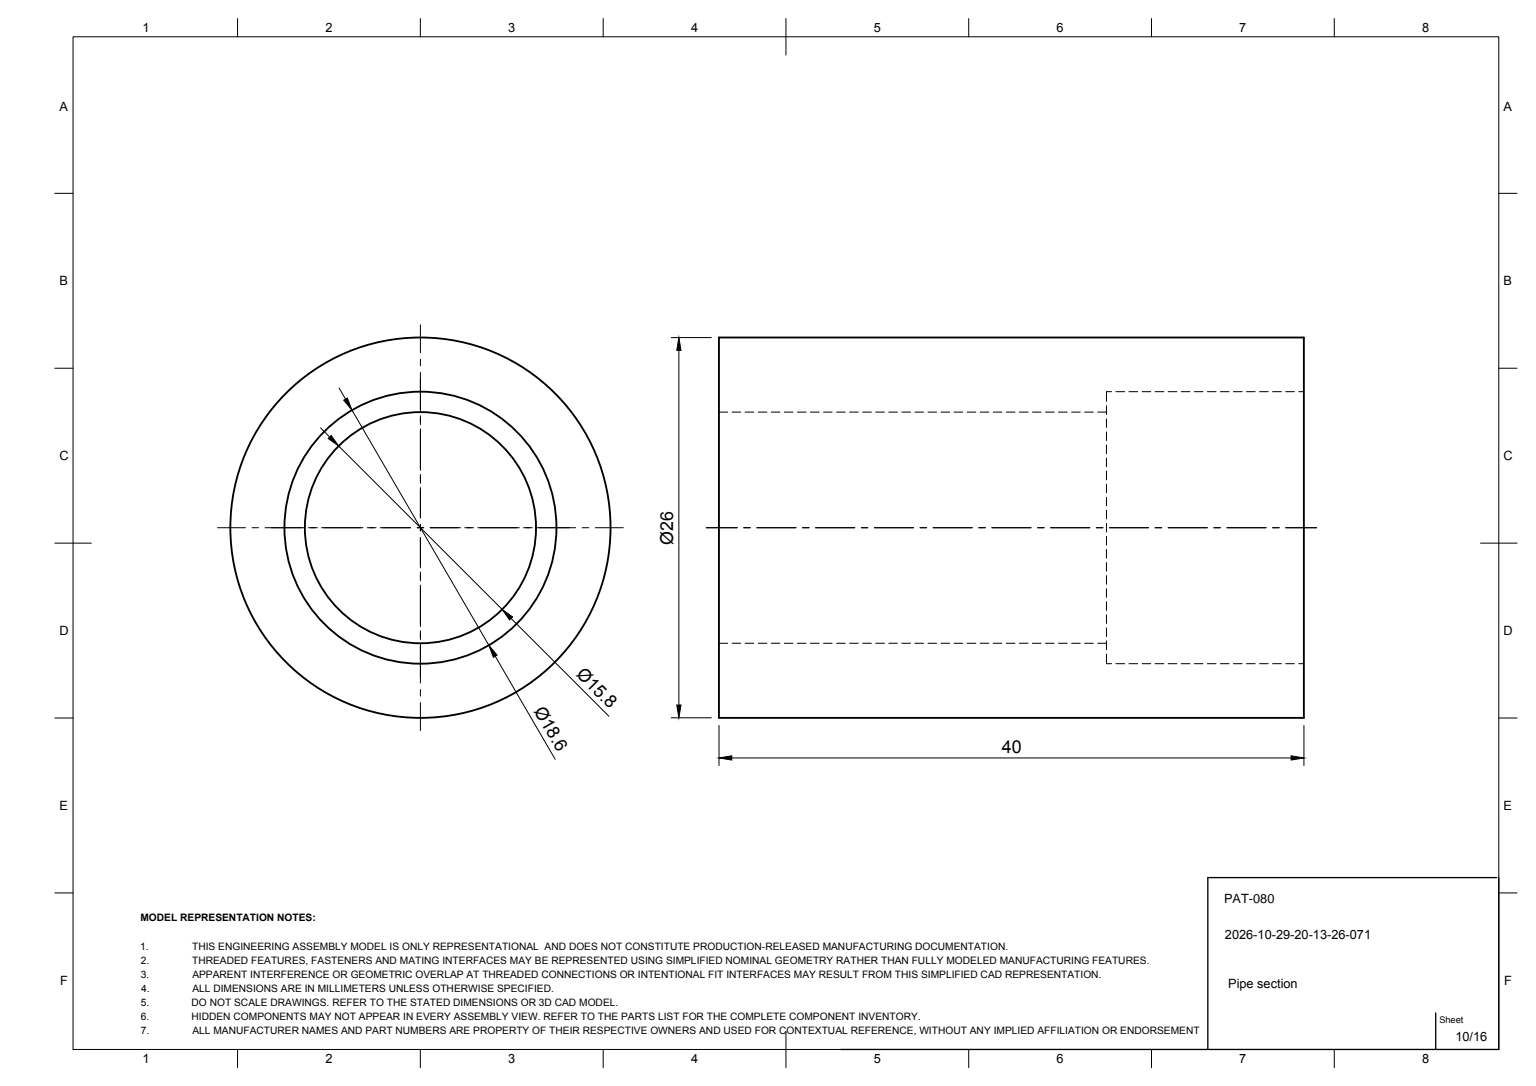
ISO-10303-21;
HEADER;
/* Generated by software containing ST-Developer
 * from STEP Tools, Inc. (www.steptools.com) 
 */

FILE_DESCRIPTION(
/* description */ ('PAT-080'),
/* implementation_level */ '2;1');

FILE_NAME(
/* name */ 'Pipe section.step',
/* time_stamp */ '2026-10-29T20:13:47-07:00',
/* author */ (''),
/* organization */ (''),
/* preprocessor_version */ 'ST-DEVELOPER v20.2',
/* originating_system */ 'Autodesk Translation Framework v15.17.0.0',
/* authorisation */ '');

FILE_SCHEMA (('AUTOMOTIVE_DESIGN { 1 0 10303 214 3 1 1 }'));
ENDSEC;

DATA;
#10=MECHANICAL_DESIGN_GEOMETRIC_PRESENTATION_REPRESENTATION('',(#253),#6878);
#215=SHAPE_REPRESENTATION_RELATIONSHIP('SRR','None',#6971,#234);
#234=ADVANCED_BREP_SHAPE_REPRESENTATION('',(#272),#6866);
#253=STYLED_ITEM('',(#7122),#272);
#272=MANIFOLD_SOLID_BREP('Body1',#3869);
#309=FACE_BOUND('',#850,.T.);
#310=FACE_BOUND('',#854,.T.);
#311=FACE_BOUND('',#856,.T.);
#427=PLANE('',#4248);
#428=PLANE('',#4255);
#429=PLANE('',#4256);
#594=FACE_OUTER_BOUND('',#848,.T.);
#595=FACE_OUTER_BOUND('',#849,.T.);
#596=FACE_OUTER_BOUND('',#851,.T.);
#597=FACE_OUTER_BOUND('',#852,.T.);
#598=FACE_OUTER_BOUND('',#853,.T.);
#599=FACE_OUTER_BOUND('',#855,.T.);
#848=EDGE_LOOP('',(#3064,#3065,#3066,#3067));
#849=EDGE_LOOP('',(#3068));
#850=EDGE_LOOP('',(#3069));
#851=EDGE_LOOP('',(#3070,#3071,#3072,#3073));
#852=EDGE_LOOP('',(#3074,#3075,#3076,#3077));
#853=EDGE_LOOP('',(#3078));
#854=EDGE_LOOP('',(#3079));
#855=EDGE_LOOP('',(#3080));
#856=EDGE_LOOP('',(#3081));
#1208=LINE('',#6216,#1523);
#1209=LINE('',#6224,#1524);
#1210=LINE('',#6229,#1525);
#1523=VECTOR('',#5020,0.93);
#1524=VECTOR('',#5031,0.79);
#1525=VECTOR('',#5036,1.3);
#1706=CIRCLE('',#4246,0.93);
#1707=CIRCLE('',#4247,0.93);
#1708=CIRCLE('',#4249,0.79);
#1709=CIRCLE('',#4251,0.79);
#1710=CIRCLE('',#4253,1.3);
#1711=CIRCLE('',#4254,1.3);
#1962=VERTEX_POINT('',#6213);
#1963=VERTEX_POINT('',#6215);
#1964=VERTEX_POINT('',#6219);
#1965=VERTEX_POINT('',#6222);
#1966=VERTEX_POINT('',#6226);
#1967=VERTEX_POINT('',#6228);
#2355=EDGE_CURVE('',#1962,#1962,#1706,.T.);
#2356=EDGE_CURVE('',#1962,#1963,#1208,.T.);
#2357=EDGE_CURVE('',#1963,#1963,#1707,.T.);
#2358=EDGE_CURVE('',#1964,#1964,#1708,.T.);
#2359=EDGE_CURVE('',#1965,#1965,#1709,.T.);
#2360=EDGE_CURVE('',#1965,#1964,#1209,.T.);
#2361=EDGE_CURVE('',#1966,#1966,#1710,.T.);
#2362=EDGE_CURVE('',#1966,#1967,#1210,.T.);
#2363=EDGE_CURVE('',#1967,#1967,#1711,.T.);
#3064=ORIENTED_EDGE('',*,*,#2355,.F.);
#3065=ORIENTED_EDGE('',*,*,#2356,.T.);
#3066=ORIENTED_EDGE('',*,*,#2357,.T.);
#3067=ORIENTED_EDGE('',*,*,#2356,.F.);
#3068=ORIENTED_EDGE('',*,*,#2357,.F.);
#3069=ORIENTED_EDGE('',*,*,#2358,.F.);
#3070=ORIENTED_EDGE('',*,*,#2359,.F.);
#3071=ORIENTED_EDGE('',*,*,#2360,.T.);
#3072=ORIENTED_EDGE('',*,*,#2358,.T.);
#3073=ORIENTED_EDGE('',*,*,#2360,.F.);
#3074=ORIENTED_EDGE('',*,*,#2361,.F.);
#3075=ORIENTED_EDGE('',*,*,#2362,.T.);
#3076=ORIENTED_EDGE('',*,*,#2363,.T.);
#3077=ORIENTED_EDGE('',*,*,#2362,.F.);
#3078=ORIENTED_EDGE('',*,*,#2361,.T.);
#3079=ORIENTED_EDGE('',*,*,#2359,.T.);
#3080=ORIENTED_EDGE('',*,*,#2363,.F.);
#3081=ORIENTED_EDGE('',*,*,#2355,.T.);
#3594=CYLINDRICAL_SURFACE('',#4245,0.93);
#3595=CYLINDRICAL_SURFACE('',#4250,0.79);
#3596=CYLINDRICAL_SURFACE('',#4252,1.3);
#3730=ADVANCED_FACE('',(#594),#3594,.F.);
#3731=ADVANCED_FACE('',(#595,#309),#427,.F.);
#3732=ADVANCED_FACE('',(#596),#3595,.F.);
#3733=ADVANCED_FACE('',(#597),#3596,.T.);
#3734=ADVANCED_FACE('',(#598,#310),#428,.T.);
#3735=ADVANCED_FACE('',(#599,#311),#429,.F.);
#3869=CLOSED_SHELL('',(#3730,#3731,#3732,#3733,#3734,#3735));
#4244=AXIS2_PLACEMENT_3D('',#6211,#5014,#5015);
#4245=AXIS2_PLACEMENT_3D('',#6212,#5016,#5017);
#4246=AXIS2_PLACEMENT_3D('',#6214,#5018,#5019);
#4247=AXIS2_PLACEMENT_3D('',#6217,#5021,#5022);
#4248=AXIS2_PLACEMENT_3D('',#6218,#5023,#5024);
#4249=AXIS2_PLACEMENT_3D('',#6220,#5025,#5026);
#4250=AXIS2_PLACEMENT_3D('',#6221,#5027,#5028);
#4251=AXIS2_PLACEMENT_3D('',#6223,#5029,#5030);
#4252=AXIS2_PLACEMENT_3D('',#6225,#5032,#5033);
#4253=AXIS2_PLACEMENT_3D('',#6227,#5034,#5035);
#4254=AXIS2_PLACEMENT_3D('',#6230,#5037,#5038);
#4255=AXIS2_PLACEMENT_3D('',#6231,#5039,#5040);
#4256=AXIS2_PLACEMENT_3D('',#6232,#5041,#5042);
#5014=DIRECTION('axis',(0.,0.,1.));
#5015=DIRECTION('refdir',(1.,0.,0.));
#5016=DIRECTION('center_axis',(1.,0.,0.));
#5017=DIRECTION('ref_axis',(0.,0.,-1.));
#5018=DIRECTION('center_axis',(1.,0.,0.));
#5019=DIRECTION('ref_axis',(0.,0.,-1.));
#5020=DIRECTION('',(1.,0.,0.));
#5021=DIRECTION('center_axis',(1.,0.,0.));
#5022=DIRECTION('ref_axis',(0.,0.,-1.));
#5023=DIRECTION('center_axis',(1.,0.,0.));
#5024=DIRECTION('ref_axis',(0.,0.,-1.));
#5025=DIRECTION('center_axis',(-1.,0.,0.));
#5026=DIRECTION('ref_axis',(0.,0.,-1.));
#5027=DIRECTION('center_axis',(1.,0.,0.));
#5028=DIRECTION('ref_axis',(0.,0.,-1.));
#5029=DIRECTION('center_axis',(-1.,0.,0.));
#5030=DIRECTION('ref_axis',(0.,0.,-1.));
#5031=DIRECTION('',(-1.,0.,0.));
#5032=DIRECTION('center_axis',(1.,0.,0.));
#5033=DIRECTION('ref_axis',(0.,0.,-1.));
#5034=DIRECTION('center_axis',(1.,0.,0.));
#5035=DIRECTION('ref_axis',(0.,0.,-1.));
#5036=DIRECTION('',(-1.,0.,0.));
#5037=DIRECTION('center_axis',(1.,0.,0.));
#5038=DIRECTION('ref_axis',(0.,0.,-1.));
#5039=DIRECTION('center_axis',(1.,0.,0.));
#5040=DIRECTION('ref_axis',(0.,0.,-1.));
#5041=DIRECTION('center_axis',(1.,0.,0.));
#5042=DIRECTION('ref_axis',(0.,0.,-1.));
#6211=CARTESIAN_POINT('',(0.,0.,0.));
#6212=CARTESIAN_POINT('Origin',(-6.9,0.,6.));
#6213=CARTESIAN_POINT('',(-6.8,-1.13892152320704E-16,6.93));
#6214=CARTESIAN_POINT('Origin',(-6.8,0.,6.));
#6215=CARTESIAN_POINT('',(-5.45,-1.13892152320704E-16,6.93));
#6216=CARTESIAN_POINT('',(-6.9,-1.13892152320704E-16,6.93));
#6217=CARTESIAN_POINT('Origin',(-5.45,0.,6.));
#6218=CARTESIAN_POINT('Origin',(-5.45,0.,6.));
#6219=CARTESIAN_POINT('',(-5.45,9.67470971326409E-17,6.79));
#6220=CARTESIAN_POINT('Origin',(-5.45,0.,6.));
#6221=CARTESIAN_POINT('Origin',(-6.8,0.,6.));
#6222=CARTESIAN_POINT('',(-2.8,-9.67470971326409E-17,6.79));
#6223=CARTESIAN_POINT('Origin',(-2.8,0.,6.));
#6224=CARTESIAN_POINT('',(-6.8,-9.67470971326409E-17,6.79));
#6225=CARTESIAN_POINT('Origin',(-6.8,0.,6.));
#6226=CARTESIAN_POINT('',(-2.8,-1.59204083889156E-16,7.3));
#6227=CARTESIAN_POINT('Origin',(-2.8,0.,6.));
#6228=CARTESIAN_POINT('',(-6.8,-1.59204083889156E-16,7.3));
#6229=CARTESIAN_POINT('',(-6.8,-1.59204083889156E-16,7.3));
#6230=CARTESIAN_POINT('Origin',(-6.8,0.,6.));
#6231=CARTESIAN_POINT('Origin',(-2.8,0.,6.));
#6232=CARTESIAN_POINT('Origin',(-6.8,0.,6.));
#6845=UNCERTAINTY_MEASURE_WITH_UNIT(LENGTH_MEASURE(0.001),#6879,
'DISTANCE_ACCURACY_VALUE',
'Maximum model space distance between geometric entities at asserted c
onnectivities');
#6857=UNCERTAINTY_MEASURE_WITH_UNIT(LENGTH_MEASURE(0.001),#6879,
'DISTANCE_ACCURACY_VALUE',
'Maximum model space distance between geometric entities at asserted c
onnectivities');
#6866=(
GEOMETRIC_REPRESENTATION_CONTEXT(3)
GLOBAL_UNCERTAINTY_ASSIGNED_CONTEXT((#6845))
GLOBAL_UNIT_ASSIGNED_CONTEXT((#6879,#6881,#6882))
REPRESENTATION_CONTEXT('','3D')
);
#6878=(
GEOMETRIC_REPRESENTATION_CONTEXT(3)
GLOBAL_UNCERTAINTY_ASSIGNED_CONTEXT((#6857))
GLOBAL_UNIT_ASSIGNED_CONTEXT((#6879,#6881,#6882))
REPRESENTATION_CONTEXT('','3D')
);
#6879=(
LENGTH_UNIT()
NAMED_UNIT(*)
SI_UNIT(.CENTI.,.METRE.)
);
#6881=(
NAMED_UNIT(*)
PLANE_ANGLE_UNIT()
SI_UNIT($,.RADIAN.)
);
#6882=(
NAMED_UNIT(*)
SI_UNIT($,.STERADIAN.)
SOLID_ANGLE_UNIT()
);
#6891=SHAPE_DEFINITION_REPRESENTATION(#6911,#6971);
#6911=PRODUCT_DEFINITION_SHAPE('',$,#6992);
#6971=SHAPE_REPRESENTATION('',(#4244),#6866);
#6983=PRODUCT_DEFINITION_CONTEXT('part definition',#7045,'design');
#6992=PRODUCT_DEFINITION('Pipe section','Pipe section',#7012,
#6983);
#7012=PRODUCT_DEFINITION_FORMATION('',$,#7055);
#7045=APPLICATION_CONTEXT(
'Core Data for Automotive Mechanical Design Process');
#7046=PRODUCT_CONTEXT('part definition',#7045,'mechanical');
#7055=PRODUCT('Pipe section','Pipe section','Pipe section',(#7046));
#7116=COLOUR_RGB('Sky Blue',0.24,0.69,0.87);
#7117=FILL_AREA_STYLE_COLOUR('',#7116);
#7118=FILL_AREA_STYLE('',(#7117));
#7119=SURFACE_STYLE_FILL_AREA(#7118);
#7120=SURFACE_SIDE_STYLE('',(#7119));
#7121=SURFACE_STYLE_USAGE(.BOTH.,#7120);
#7122=PRESENTATION_STYLE_ASSIGNMENT((#7121));
ENDSEC;
END-ISO-10303-21;
